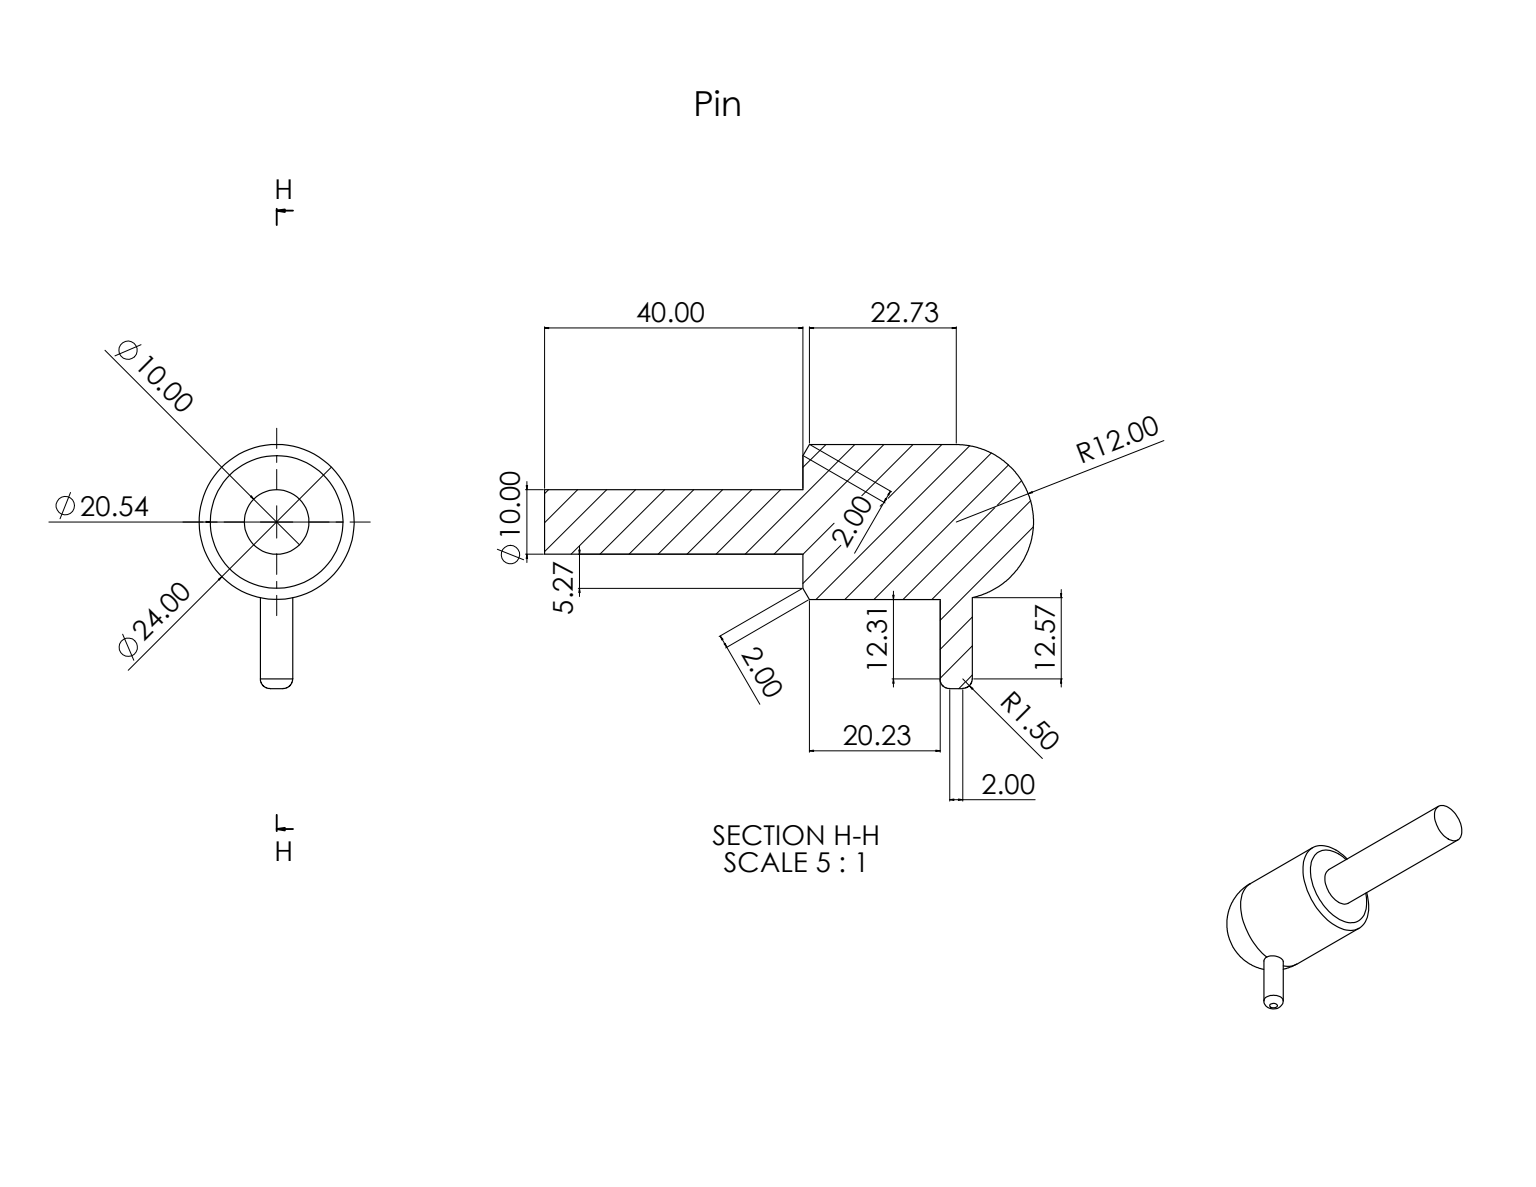
ISO-10303-21;
HEADER;
FILE_DESCRIPTION (('STEP AP214'),
    '1' );
FILE_NAME ('Pin.step',
    '2026-10-26T22:46:44',
    ( '' ),
    ( '' ),
    'SwSTEP 2.0',
    'SolidWorks 2025',
    '' );
FILE_SCHEMA (( 'AUTOMOTIVE_DESIGN' ));
ENDSEC;

DATA;
#9=ORIENTED_EDGE ( 'NONE', *, *, #6510, .F. ) ;
#38=VERTEX_POINT ( 'NONE', #5675 ) ;
#116=DIRECTION ( 'NONE',  ( -0.8660254037844363761, -0.5000000000000043299, 6.872020471724002955E-17 ) ) ;
#132=ORIENTED_EDGE ( 'NONE', *, *, #6398, .F. ) ;
#195=EDGE_CURVE ( 'NONE', #20338, #18465, #2729, .T. ) ;
#229=DIRECTION ( 'NONE',  ( -0.5000000000000046629, 0.8660254037844360431, -0.000000000000000000 ) ) ;
#280=EDGE_LOOP ( 'NONE', ( #9635, #17921, #8883, #13281 ) ) ;
#349=AXIS2_PLACEMENT_3D ( 'NONE', #19014, #17316, #10832 ) ;
#381=ORIENTED_EDGE ( 'NONE', *, *, #17715, .T. ) ;
#391=CIRCLE ( 'NONE', #14642, 12.00000000000002665 ) ;
#499=CARTESIAN_POINT ( 'NONE',  ( 105.1989074543211871, 189.2062061502930135, 11.00000000000001066 ) ) ;
#500=CARTESIAN_POINT ( 'NONE',  ( 97.86136863954072851, 199.4073499008320027, 8.831051211850477145 ) ) ;
#557=ADVANCED_FACE ( 'NONE', ( #8943 ), #5256, .T. ) ;
#571=( NAMED_UNIT ( * ) PLANE_ANGLE_UNIT ( ) SI_UNIT ( $, .RADIAN. ) );
#573=VECTOR ( 'NONE', #13152, 1000.000000000000000 ) ;
#597=DIRECTION ( 'NONE',  ( 0.5000000000000046629, -0.8660254037844360431, 0.000000000000000000 ) ) ;
#619=VECTOR ( 'NONE', #4263, 1000.000000000000114 ) ;
#670=DIRECTION ( 'NONE',  ( 0.8660254037844362651, 0.5000000000000042188, -6.872020471724000490E-17 ) ) ;
#680=AXIS2_PLACEMENT_3D ( 'NONE', #1042, #9181, #2945 ) ;
#733=ORIENTED_EDGE ( 'NONE', *, *, #2224, .T. ) ;
#738=ORIENTED_EDGE ( 'NONE', *, *, #7937, .F. ) ;
#748=AXIS2_PLACEMENT_3D ( 'NONE', #7309, #8909, #2142 ) ;
#770=VECTOR ( 'NONE', #5873, 1000.000000000000000 ) ;
#808=CARTESIAN_POINT ( 'NONE',  ( 96.97892280296886724, 198.7003685781201057, 10.19262075797938749 ) ) ;
#850=CARTESIAN_POINT ( 'NONE',  ( 93.04593889385130012, 210.2557651598135351, 11.00000000000001066 ) ) ;
#883=FACE_BOUND ( 'NONE', #17859, .T. ) ;
#886=DIRECTION ( 'NONE',  ( 0.5000000000000045519, -0.8660254037844359321, 0.000000000000000000 ) ) ;
#911=CARTESIAN_POINT ( 'NONE',  ( 98.22805148513273821, 199.6643403035069753, 8.628462948306966140 ) ) ;
#938=EDGE_LOOP ( 'NONE', ( #1013, #381, #3588, #9, #15721 ) ) ;
#1013=ORIENTED_EDGE ( 'NONE', *, *, #3059, .T. ) ;
#1042=CARTESIAN_POINT ( 'NONE',  ( 106.0649328581056210, 189.7062061502930135, 11.00000000000001066 ) ) ;
#1091=CARTESIAN_POINT ( 'NONE',  ( 105.9489074543212013, 187.9071680446163555, 11.00000000000001066 ) ) ;
#1274=DIRECTION ( 'NONE',  ( 0.000000000000000000, 0.000000000000000000, 1.000000000000000000 ) ) ;
#1345=VERTEX_POINT ( 'NONE', #2130 ) ;
#1356=CARTESIAN_POINT ( 'NONE',  ( 96.89336873520835525, 198.6246579379146340, 11.32949238779788637 ) ) ;
#1392=ORIENTED_EDGE ( 'NONE', *, *, #8590, .F. ) ;
#1422=ORIENTED_EDGE ( 'NONE', *, *, #8317, .T. ) ;
#1435=ORIENTED_EDGE ( 'NONE', *, *, #6398, .T. ) ;
#1450=ADVANCED_FACE ( 'NONE', ( #16963 ), #5914, .T. ) ;
#1455=VERTEX_POINT ( 'NONE', #2551 ) ;
#1460=CARTESIAN_POINT ( 'NONE',  ( 98.91428619100412334, 200.0914894846854679, 13.49999999999996803 ) ) ;
#1469=DIRECTION ( 'NONE',  ( 0.5000000000000046629, -0.8660254037844360431, 0.000000000000000000 ) ) ;
#1562=CARTESIAN_POINT ( 'NONE',  ( 97.35757311143078141, 199.0198733241707600, 12.65155119472265710 ) ) ;
#1569=ORIENTED_EDGE ( 'NONE', *, *, #8317, .F. ) ;
#1666=CARTESIAN_POINT ( 'NONE',  ( 73.36131599811851345, 198.8908428320658288, 11.00000000000001066 ) ) ;
#1667=CARTESIAN_POINT ( 'NONE',  ( 98.62918417965860840, 199.9227537566937940, 13.48335911653028596 ) ) ;
#1681=ORIENTED_EDGE ( 'NONE', *, *, #3937, .T. ) ;
#1704=MECHANICAL_DESIGN_GEOMETRIC_PRESENTATION_REPRESENTATION('',(#5407),#9480);
#1731=AXIS2_PLACEMENT_3D ( 'NONE', #16410, #12923, #9813 ) ;
#1929=CARTESIAN_POINT ( 'NONE',  ( 67.36131599811849924, 207.2831476774790076, 11.00000000000001066 ) ) ;
#2004=DIRECTION ( 'NONE',  ( -0.8660254037844380415, -0.5000000000000008882, 0.000000000000000000 ) ) ;
#2024=DIRECTION ( 'NONE',  ( 0.5000000000000044409, -0.8660254037844360431, 0.000000000000000000 ) ) ;
#2072=AXIS2_PLACEMENT_3D ( 'NONE', #14737, #11324, #13027 ) ;
#2086=CARTESIAN_POINT ( 'NONE',  ( 98.36082807960120533, 199.7525165975381469, 8.580140356014970493 ) ) ;
#2130=CARTESIAN_POINT ( 'NONE',  ( 74.99529059433412215, 194.0607158131436165, 11.00000000000001066 ) ) ;
#2142=DIRECTION ( 'NONE',  ( 0.5000000000000047740, -0.8660254037844359321, 0.000000000000000000 ) ) ;
#2181=AXIS2_PLACEMENT_3D ( 'NONE', #850, #7300, #2761 ) ;
#2224=EDGE_CURVE ( 'NONE', #13549, #1455, #17632, .T. ) ;
#2258=DIRECTION ( 'NONE',  ( -0.8660254037844363761, -0.5000000000000043299, 6.872020471724002955E-17 ) ) ;
#2370=DIRECTION ( 'NONE',  ( -0.8660254037844363761, -0.5000000000000043299, 6.872020471724002955E-17 ) ) ;
#2531=ADVANCED_FACE ( 'NONE', ( #3362 ), #12924, .T. ) ;
#2551=CARTESIAN_POINT ( 'NONE',  ( 77.62926519054968821, 189.4985379866525648, 11.00000000000001066 ) ) ;
#2596=VERTEX_POINT ( 'NONE', #16411 ) ;
#2718=LINE ( 'NONE', #18403, #770 ) ;
#2729=LINE ( 'NONE', #17243, #19805 ) ;
#2757=TOROIDAL_SURFACE ( 'NONE', #11894, 0.9999999999999974465, 1.500000000000000000 ) ;
#2761=DIRECTION ( 'NONE',  ( 0.5000000000000039968, -0.8660254037844362651, 0.000000000000000000 ) ) ;
#2793=AXIS2_PLACEMENT_3D ( 'NONE', #10566, #15166, #13557 ) ;
#2824=DIRECTION ( 'NONE',  ( -0.8660254037844380415, -0.5000000000000008882, 0.000000000000000000 ) ) ;
#2902=FACE_OUTER_BOUND ( 'NONE', #938, .T. ) ;
#2909=DIRECTION ( 'NONE',  ( 0.5000000000000046629, -0.8660254037844360431, 0.000000000000000000 ) ) ;
#2945=DIRECTION ( 'NONE',  ( -1.000000000000000000, 0.000000000000000000, 0.000000000000000000 ) ) ;
#2954=ORIENTED_EDGE ( 'NONE', *, *, #13976, .T. ) ;
#3029=CARTESIAN_POINT ( 'NONE',  ( 98.91428619100412334, 200.0914894846854679, 8.500000000000049738 ) ) ;
#3038=AXIS2_PLACEMENT_3D ( 'NONE', #9596, #11629, #9905 ) ;
#3059=EDGE_CURVE ( 'NONE', #13220, #13875, #391, .T. ) ;
#3151=CARTESIAN_POINT ( 'NONE',  ( 97.07523654288182513, 198.7838771924956518, 12.10917801131580163 ) ) ;
#3155=CARTESIAN_POINT ( 'NONE',  ( 101.0793497004652863, 201.3414894846855248, 11.00000000000001066 ) ) ;
#3221=FACE_OUTER_BOUND ( 'NONE', #4011, .T. ) ;
#3246=CARTESIAN_POINT ( 'NONE',  ( 97.54126021093399856, 199.1658384139430495, 12.88365451894100389 ) ) ;
#3352=CARTESIAN_POINT ( 'NONE',  ( 96.97854020012087517, 198.7000365498672920, 11.80616005232970345 ) ) ;
#3362=FACE_OUTER_BOUND ( 'NONE', #13334, .T. ) ;
#3376=ORIENTED_EDGE ( 'NONE', *, *, #13981, .T. ) ;
#3399=DIRECTION ( 'NONE',  ( 0.8660254037844380415, 0.5000000000000008882, 0.000000000000000000 ) ) ;
#3422=EDGE_CURVE ( 'NONE', #1455, #2596, #2718, .T. ) ;
#3504=DIRECTION ( 'NONE',  ( 0.8660254037844360431, 0.5000000000000045519, 0.000000000000000000 ) ) ;
#3557=CARTESIAN_POINT ( 'NONE',  ( 72.49529059433406530, 198.3908428320658288, 11.00000000000001066 ) ) ;
#3588=ORIENTED_EDGE ( 'NONE', *, *, #12543, .T. ) ;
#3632=CARTESIAN_POINT ( 'NONE',  ( 69.99529059433403688, 202.7209698509880411, 11.00000000000001066 ) ) ;
#3738=DIRECTION ( 'NONE',  ( 0.5000000000000047740, -0.8660254037844359321, 0.000000000000000000 ) ) ;
#3811=MANIFOLD_SOLID_BREP ( 'Chamfer2', #17459 ) ;
#3819=VERTEX_POINT ( 'NONE', #18382 ) ;
#3860=EDGE_CURVE ( 'NONE', #6967, #13875, #6093, .T. ) ;
#3872=CARTESIAN_POINT ( 'NONE',  ( 98.63149783568741213, 199.9241707403680834, 8.516312532717298822 ) ) ;
#3937=EDGE_CURVE ( 'NONE', #18465, #13223, #17962, .T. ) ;
#3956=DIRECTION ( 'NONE',  ( 0.8660254037844380415, 0.5000000000000008882, 0.000000000000000000 ) ) ;
#3984=DIRECTION ( 'NONE',  ( -0.8660254037844361541, -0.5000000000000042188, 6.872020471724001723E-17 ) ) ;
#4011=EDGE_LOOP ( 'NONE', ( #7091, #9421, #18763, #7287 ) ) ;
#4028=CARTESIAN_POINT ( 'NONE',  ( 73.36131599811851345, 198.8908428320658288, 11.00000000000001066 ) ) ;
#4062=ORIENTED_EDGE ( 'NONE', *, *, #3059, .F. ) ;
#4063=AXIS2_PLACEMENT_3D ( 'NONE', #11056, #9339, #886 ) ;
#4138=CONICAL_SURFACE ( 'NONE', #12604, 10.26794919243114634, 1.047197551196596965 ) ;
#4263=DIRECTION ( 'NONE',  ( -0.8660254037844362651, -0.5000000000000042188, 6.872020471724002955E-17 ) ) ;
#4331=AXIS2_PLACEMENT_3D ( 'NONE', #18797, #670, #19952 ) ;
#4359=VERTEX_POINT ( 'NONE', #3155 ) ;
#4366=LINE ( 'NONE', #18896, #619 ) ;
#4402=CIRCLE ( 'NONE', #6404, 5.000000000000039968 ) ;
#4417=AXIS2_PLACEMENT_3D ( 'NONE', #10195, #16577, #3956 ) ;
#4590=DIRECTION ( 'NONE',  ( -0.8660254037844363761, -0.5000000000000043299, 6.872020471724002955E-17 ) ) ;
#4591=FACE_OUTER_BOUND ( 'NONE', #12229, .T. ) ;
#4660=CARTESIAN_POINT ( 'NONE',  ( 98.91428619100422281, 200.0914894846855248, 11.00000000000001066 ) ) ;
#4681=CARTESIAN_POINT ( 'NONE',  ( 103.4382437392645642, 216.2557651598135919, 11.00000000000001066 ) ) ;
#4910=DIRECTION ( 'NONE',  ( 0.8660254037844360431, 0.5000000000000045519, 0.000000000000000000 ) ) ;
#4997=EDGE_CURVE ( 'NONE', #11555, #17136, #5615, .T. ) ;
#5036=DIRECTION ( 'NONE',  ( -0.8660254037844363761, -0.5000000000000043299, 6.872020471724002955E-17 ) ) ;
#5075=AXIS2_PLACEMENT_3D ( 'NONE', #11592, #2258, #15212 ) ;
#5112=EDGE_CURVE ( 'NONE', #1455, #13549, #11532, .T. ) ;
#5132=ORIENTED_EDGE ( 'NONE', *, *, #5112, .T. ) ;
#5166=CARTESIAN_POINT ( 'NONE',  ( 93.04593889385130012, 210.2557651598135351, 11.00000000000000888 ) ) ;
#5185=FACE_OUTER_BOUND ( 'NONE', #16023, .T. ) ;
#5256=TOROIDAL_SURFACE ( 'NONE', #16125, 0.9999999999999974465, 1.500000000000000000 ) ;
#5277=AXIS2_PLACEMENT_3D ( 'NONE', #5556, #3984, #16817 ) ;
#5343=AXIS2_PLACEMENT_3D ( 'NONE', #19222, #20589, #19320 ) ;
#5404=ORIENTED_EDGE ( 'NONE', *, *, #3422, .F. ) ;
#5407=STYLED_ITEM('',(#20988),#3811);
#5445=CARTESIAN_POINT ( 'NONE',  ( 97.26699134085764342, 198.9478798014807808, 9.463061291710214817 ) ) ;
#5500=DIRECTION ( 'NONE',  ( -0.5000000000000043299, 0.8660254037844360431, 0.000000000000000000 ) ) ;
#5556=CARTESIAN_POINT ( 'NONE',  ( 37.85427444295662269, 178.3908428320656299, 11.00000000000001243 ) ) ;
#5576=FACE_OUTER_BOUND ( 'NONE', #13860, .T. ) ;
#5615=LINE ( 'NONE', #12210, #7450 ) ;
#5639=EDGE_CURVE ( 'NONE', #17136, #3819, #6442, .T. ) ;
#5648=( NAMED_UNIT ( * ) PLANE_ANGLE_UNIT ( ) SI_UNIT ( $, .RADIAN. ) );
#5675=CARTESIAN_POINT ( 'NONE',  ( 67.36131599811847082, 209.2831476774790360, 11.00000000000001066 ) ) ;
#5804=ORIENTED_EDGE ( 'NONE', *, *, #195, .F. ) ;
#5824=DIRECTION ( 'NONE',  ( -0.8660254037844362651, -0.5000000000000042188, 6.872020471724002955E-17 ) ) ;
#5837=ORIENTED_EDGE ( 'NONE', *, *, #16586, .T. ) ;
#5864=ADVANCED_FACE ( 'NONE', ( #3221 ), #4138, .T. ) ;
#5873=DIRECTION ( 'NONE',  ( 0.8660254037844417052, -0.4999999999999947820, 1.060575238724906422E-16 ) ) ;
#5914=SPHERICAL_SURFACE ( 'NONE', #2181, 12.00000000000002665 ) ;
#5939=DIRECTION ( 'NONE',  ( 0.5000000000000046629, -0.8660254037844360431, 0.000000000000000000 ) ) ;
#6062=ORIENTED_EDGE ( 'NONE', *, *, #8091, .T. ) ;
#6093=CIRCLE ( 'NONE', #349, 12.00000000000002487 ) ;
#6207=DIRECTION ( 'NONE',  ( 0.8660254037844380415, 0.5000000000000008882, 0.000000000000000000 ) ) ;
#6292=ORIENTED_EDGE ( 'NONE', *, *, #5639, .T. ) ;
#6337=CARTESIAN_POINT ( 'NONE',  ( 87.04593889385124328, 220.6480700052267707, 11.00000000000001066 ) ) ;
#6398=EDGE_CURVE ( 'NONE', #1345, #20338, #18340, .T. ) ;
#6404=AXIS2_PLACEMENT_3D ( 'NONE', #3557, #5036, #14722 ) ;
#6409=DIRECTION ( 'NONE',  ( -0.5000000000000046629, 0.8660254037844360431, -0.000000000000000000 ) ) ;
#6411=CARTESIAN_POINT ( 'NONE',  ( 96.94231704718730214, 198.6680486871722167, 11.65021776913269314 ) ) ;
#6442=CIRCLE ( 'NONE', #1731, 1.500000000000001332 ) ;
#6466=B_SPLINE_CURVE_WITH_KNOTS ( 'NONE', 3,
 ( #7701, #12805, #1356, #6411, #3352, #3151, #16095, #11311, #1562, #3246, #12702, #14307, #16195, #20741, #19060, #1667, #19161, #1460 ),
 .UNSPECIFIED., .F., .F.,
 ( 4, 2, 2, 2, 2, 2, 2, 2, 4 ),
 ( 0.003919784392900028426, 0.004409243773870153045, 0.004898703154840278531, 0.005388162535810403150, 0.005877621916780527769, 0.006367081297750653256, 0.006856540678720777875, 0.007346000059690903361, 0.007835459440661027980 ),
 .UNSPECIFIED. ) ;
#6510=EDGE_CURVE ( 'NONE', #11555, #2596, #12726, .T. ) ;
#6558=CYLINDRICAL_SURFACE ( 'NONE', #7051, 5.000000000000036415 ) ;
#6588=CIRCLE ( 'NONE', #19472, 0.9999999999999917843 ) ;
#6652=DIRECTION ( 'NONE',  ( -0.5000000000000045519, 0.8660254037844359321, 0.000000000000000000 ) ) ;
#6688=ADVANCED_FACE ( 'NONE', ( #13531 ), #2757, .T. ) ;
#6715=VECTOR ( 'NONE', #16730, 1000.000000000000114 ) ;
#6805=EDGE_LOOP ( 'NONE', ( #16956, #13022, #20421, #17398, #20769 ) ) ;
#6825=VECTOR ( 'NONE', #5824, 1000.000000000000114 ) ;
#6967=VERTEX_POINT ( 'NONE', #4681 ) ;
#7051=AXIS2_PLACEMENT_3D ( 'NONE', #8259, #7854, #19304 ) ;
#7091=ORIENTED_EDGE ( 'NONE', *, *, #5112, .F. ) ;
#7098=LINE ( 'NONE', #19815, #10331 ) ;
#7148=EDGE_CURVE ( 'NONE', #17136, #10069, #20322, .T. ) ;
#7154=CARTESIAN_POINT ( 'NONE',  ( 97.97831163141611910, 199.4916918115227702, 8.754184836083465981 ) ) ;
#7258=CARTESIAN_POINT ( 'NONE',  ( 96.89297785063146762, 198.6243099879737599, 10.67381219715677609 ) ) ;
#7270=CARTESIAN_POINT ( 'NONE',  ( 103.0338439448600951, 187.9562061502930135, 11.00000000000001066 ) ) ;
#7287=ORIENTED_EDGE ( 'NONE', *, *, #16586, .F. ) ;
#7300=DIRECTION ( 'NONE',  ( 5.951344303839691563E-17, 3.436010235862028595E-17, 1.000000000000000000 ) ) ;
#7309=CARTESIAN_POINT ( 'NONE',  ( 72.49529059433406530, 198.3908428320658288, 11.00000000000001066 ) ) ;
#7378=( GEOMETRIC_REPRESENTATION_CONTEXT ( 3 ) GLOBAL_UNCERTAINTY_ASSIGNED_CONTEXT ( ( #20801 ) ) GLOBAL_UNIT_ASSIGNED_CONTEXT ( ( #20084, #5648, #15029 ) ) REPRESENTATION_CONTEXT ( 'NONE', 'WORKASPACE' ) );
#7429=AXIS2_PLACEMENT_3D ( 'NONE', #1666, #8005, #12910 ) ;
#7450=VECTOR ( 'NONE', #20360, 1000.000000000000227 ) ;
#7624=CARTESIAN_POINT ( 'NONE',  ( 107.3639709637822648, 190.4562061502930135, 11.00000000000001066 ) ) ;
#7645=DIRECTION ( 'NONE',  ( 0.8660254037844360431, 0.5000000000000045519, 0.000000000000000000 ) ) ;
#7661=ORIENTED_EDGE ( 'NONE', *, *, #7148, .T. ) ;
#7698=DIRECTION ( 'NONE',  ( 0.8660254037844380415, 0.5000000000000008882, 0.000000000000000000 ) ) ;
#7701=CARTESIAN_POINT ( 'NONE',  ( 96.88087538439037871, 198.6134603144003563, 11.00000000000000888 ) ) ;
#7741=EDGE_CURVE ( 'NONE', #10069, #7744, #13554, .T. ) ;
#7744=VERTEX_POINT ( 'NONE', #20740 ) ;
#7802=FACE_OUTER_BOUND ( 'NONE', #6805, .T. ) ;
#7854=DIRECTION ( 'NONE',  ( -0.8660254037844361541, -0.5000000000000042188, 6.872020471724001723E-17 ) ) ;
#7902=EDGE_CURVE ( 'NONE', #20338, #1345, #4402, .T. ) ;
#7937=EDGE_CURVE ( 'NONE', #2596, #38, #20300, .T. ) ;
#7976=EDGE_CURVE ( 'NONE', #6967, #4359, #9123, .T. ) ;
#8005=DIRECTION ( 'NONE',  ( 0.8660254037844360431, 0.5000000000000045519, 0.000000000000000000 ) ) ;
#8091=EDGE_CURVE ( 'NONE', #10891, #11555, #13948, .T. ) ;
#8131=AXIS2_PLACEMENT_3D ( 'NONE', #8265, #229, #3399 ) ;
#8259=CARTESIAN_POINT ( 'NONE',  ( 37.85427444295662269, 178.3908428320656299, 11.00000000000001243 ) ) ;
#8265=CARTESIAN_POINT ( 'NONE',  ( 105.1989074543211728, 189.2062061502930135, 11.00000000000001066 ) ) ;
#8271=ORIENTED_EDGE ( 'NONE', *, *, #13981, .F. ) ;
#8285=EDGE_LOOP ( 'NONE', ( #20903, #12020, #4062, #1422 ) ) ;
#8289=CARTESIAN_POINT ( 'NONE',  ( 72.49529059433407951, 198.3908428320658288, 11.00000000000001066 ) ) ;
#8317=EDGE_CURVE ( 'NONE', #13220, #4359, #9469, .T. ) ;
#8507=ADVANCED_FACE ( 'NONE', ( #10087 ), #19750, .T. ) ;
#8590=EDGE_CURVE ( 'NONE', #13223, #18465, #18287, .T. ) ;
#8644=CARTESIAN_POINT ( 'NONE',  ( 98.77077497239712045, 200.0086332439910279, 8.500000000000021316 ) ) ;
#8650=AXIS2_PLACEMENT_3D ( 'NONE', #12090, #3504, #5500 ) ;
#8687=ADVANCED_FACE ( 'NONE', ( #4591 ), #19016, .T. ) ;
#8732=DIRECTION ( 'NONE',  ( 0.5000000000000038858, -0.8660254037844362651, 0.000000000000000000 ) ) ;
#8746=CARTESIAN_POINT ( 'NONE',  ( 98.91428619100412334, 200.0914894846854679, 13.49999999999996803 ) ) ;
#8883=ORIENTED_EDGE ( 'NONE', *, *, #7741, .T. ) ;
#8899=PRODUCT_DEFINITION_SHAPE ( 'NONE', 'NONE',  #10936 ) ;
#8909=DIRECTION ( 'NONE',  ( -0.8660254037844363761, -0.5000000000000043299, 6.872020471724002955E-17 ) ) ;
#8932=( LENGTH_UNIT ( ) NAMED_UNIT ( * ) SI_UNIT ( .MILLI., .METRE. ) );
#8943=FACE_OUTER_BOUND ( 'NONE', #280, .T. ) ;
#9095=PLANE ( 'NONE',  #17863 ) ;
#9123=CIRCLE ( 'NONE', #3038, 12.00000000000002487 ) ;
#9127=CARTESIAN_POINT ( 'NONE',  ( 40.35427444295665822, 174.0607158131434176, 11.00000000000001243 ) ) ;
#9139=AXIS2_PLACEMENT_3D ( 'NONE', #13619, #2370, #3738 ) ;
#9181=DIRECTION ( 'NONE',  ( 0.000000000000000000, 0.000000000000000000, -1.000000000000000000 ) ) ;
#9236=CARTESIAN_POINT ( 'NONE',  ( 37.85427444295662269, 178.3908428320656299, 11.00000000000001243 ) ) ;
#9280=CARTESIAN_POINT ( 'NONE',  ( 105.1989074543211728, 189.2062061502930135, 11.00000000000001066 ) ) ;
#9339=DIRECTION ( 'NONE',  ( -0.8660254037844361541, -0.5000000000000042188, 6.872020471724001723E-17 ) ) ;
#9351=UNCERTAINTY_MEASURE_WITH_UNIT (LENGTH_MEASURE( 1.000000000000000082E-05 ), #8932, 'distance_accuracy_value', 'NONE');
#9421=ORIENTED_EDGE ( 'NONE', *, *, #3422, .T. ) ;
#9469=CIRCLE ( 'NONE', #19640, 2.499999999999997780 ) ;
#9480=( GEOMETRIC_REPRESENTATION_CONTEXT ( 3 ) GLOBAL_UNCERTAINTY_ASSIGNED_CONTEXT ( ( #9351 ) ) GLOBAL_UNIT_ASSIGNED_CONTEXT ( ( #8932, #571, #12122 ) ) REPRESENTATION_CONTEXT ( 'NONE', 'WORKASPACE' ) );
#9596=CARTESIAN_POINT ( 'NONE',  ( 93.04593889385130012, 210.2557651598135351, 11.00000000000001066 ) ) ;
#9635=ORIENTED_EDGE ( 'NONE', *, *, #5639, .F. ) ;
#9672=AXIS2_PLACEMENT_3D ( 'NONE', #4660, #14541, #2004 ) ;
#9676=DIRECTION ( 'NONE',  ( -0.5000000000000043299, 0.8660254037844360431, 0.000000000000000000 ) ) ;
#9782=ORIENTED_EDGE ( 'NONE', *, *, #7741, .F. ) ;
#9795=ORIENTED_EDGE ( 'NONE', *, *, #3860, .F. ) ;
#9806=CYLINDRICAL_SURFACE ( 'NONE', #5277, 5.000000000000036415 ) ;
#9813=DIRECTION ( 'NONE',  ( 1.000000000000000000, 0.000000000000000000, 0.000000000000000000 ) ) ;
#9855=CIRCLE ( 'NONE', #14973, 0.9999999999999917843 ) ;
#9905=DIRECTION ( 'NONE',  ( -1.000000000000000000, 0.000000000000000000, 0.000000000000000000 ) ) ;
#9948=EDGE_LOOP ( 'NONE', ( #19226, #6292, #11319, #9782 ) ) ;
#10069=VERTEX_POINT ( 'NONE', #7624 ) ;
#10087=FACE_OUTER_BOUND ( 'NONE', #12180, .T. ) ;
#10109=DIRECTION ( 'NONE',  ( 0.8660254037844359321, 0.5000000000000046629, 0.000000000000000000 ) ) ;
#10195=CARTESIAN_POINT ( 'NONE',  ( 94.31531706421118599, 208.0571376747316492, 11.00000000000001066 ) ) ;
#10331=VECTOR ( 'NONE', #2024, 1000.000000000000227 ) ;
#10344=CIRCLE ( 'NONE', #9672, 2.499999999999997780 ) ;
#10370=ADVANCED_FACE ( 'NONE', ( #5576 ), #15061, .T. ) ;
#10420=SHAPE_REPRESENTATION_RELATIONSHIP ( 'NONE' , 'NONE' ,  #14136, #12645 ) ;
#10456=EDGE_LOOP ( 'NONE', ( #733, #5132 ) ) ;
#10566=CARTESIAN_POINT ( 'NONE',  ( 105.9489074543212013, 187.9071680446163555, 11.00000000000001066 ) ) ;
#10643=DIRECTION ( 'NONE',  ( -0.5000000000000037748, 0.8660254037844364872, 0.000000000000000000 ) ) ;
#10653=DIRECTION ( 'NONE',  ( -0.8660254037844362651, -0.5000000000000042188, 6.872020471724002955E-17 ) ) ;
#10832=DIRECTION ( 'NONE',  ( 1.000000000000000000, 0.000000000000000000, -1.445602896647336205E-16 ) ) ;
#10891=VERTEX_POINT ( 'NONE', #3029 ) ;
#10936=PRODUCT_DEFINITION ( 'UNKNOWN', '', #18249, #14271 ) ;
#11028=CARTESIAN_POINT ( 'NONE',  ( 43.85427444295667954, 167.9985379866523942, 11.00000000000001243 ) ) ;
#11051=AXIS2_PLACEMENT_3D ( 'NONE', #5166, #18219, #18017 ) ;
#11056=CARTESIAN_POINT ( 'NONE',  ( 37.85427444295662269, 178.3908428320656299, 11.00000000000001243 ) ) ;
#11264=CIRCLE ( 'NONE', #17700, 12.00000000000000178 ) ;
#11270=DIRECTION ( 'NONE',  ( 0.5000000000000047740, -0.8660254037844359321, 0.000000000000000000 ) ) ;
#11311=CARTESIAN_POINT ( 'NONE',  ( 97.27623782526788432, 198.9531532459614880, 12.52486517255494824 ) ) ;
#11319=ORIENTED_EDGE ( 'NONE', *, *, #14796, .F. ) ;
#11324=DIRECTION ( 'NONE',  ( 5.951344303839691563E-17, 3.436010235862028595E-17, 1.000000000000000000 ) ) ;
#11352=FACE_OUTER_BOUND ( 'NONE', #15794, .T. ) ;
#11445=EDGE_CURVE ( 'NONE', #3819, #7744, #9855, .T. ) ;
#11532=CIRCLE ( 'NONE', #16270, 10.26794919243111437 ) ;
#11555=VERTEX_POINT ( 'NONE', #16409 ) ;
#11592=CARTESIAN_POINT ( 'NONE',  ( 72.49529059433409373, 198.3908428320658004, 11.00000000000001066 ) ) ;
#11629=DIRECTION ( 'NONE',  ( -5.951344303839690331E-17, -3.436010235862032909E-17, -1.000000000000000000 ) ) ;
#11690=ORIENTED_EDGE ( 'NONE', *, *, #4997, .T. ) ;
#11791=ORIENTED_EDGE ( 'NONE', *, *, #7937, .T. ) ;
#11894=AXIS2_PLACEMENT_3D ( 'NONE', #499, #597, #10109 ) ;
#11927=CARTESIAN_POINT ( 'NONE',  ( 93.04593889385130012, 210.2557651598135351, 11.00000000000000888 ) ) ;
#11945=CARTESIAN_POINT ( 'NONE',  ( 96.88087538439039292, 198.6134603144004132, 10.83638872456144675 ) ) ;
#11963=CIRCLE ( 'NONE', #14686, 2.499999999999997780 ) ;
#11975=AXIS2_PLACEMENT_3D ( 'NONE', #14304, #20739, #6207 ) ;
#12020=ORIENTED_EDGE ( 'NONE', *, *, #3860, .T. ) ;
#12031=DIRECTION ( 'NONE',  ( -0.8660254037844363761, -0.5000000000000043299, 6.872020471724002955E-17 ) ) ;
#12090=CARTESIAN_POINT ( 'NONE',  ( 72.49529059433407951, 198.3908428320658288, 11.00000000000001066 ) ) ;
#12120=FACE_OUTER_BOUND ( 'NONE', #10456, .T. ) ;
#12122=( NAMED_UNIT ( * ) SI_UNIT ( $, .STERADIAN. ) SOLID_ANGLE_UNIT ( ) );
#12180=EDGE_LOOP ( 'NONE', ( #18941, #11690, #7661, #19069, #1569 ) ) ;
#12188=DIRECTION ( 'NONE',  ( -0.5000000000000042188, 0.8660254037844362651, 0.000000000000000000 ) ) ;
#12210=CARTESIAN_POINT ( 'NONE',  ( 92.15025355475009405, 206.8071376747316492, 11.00000000000001066 ) ) ;
#12229=EDGE_LOOP ( 'NONE', ( #17533, #3376, #6062, #13729, #11791 ) ) ;
#12248=DIRECTION ( 'NONE',  ( 0.8660254037844359321, 0.5000000000000046629, 0.000000000000000000 ) ) ;
#12308=FACE_OUTER_BOUND ( 'NONE', #15169, .T. ) ;
#12543=EDGE_CURVE ( 'NONE', #38, #2596, #11264, .T. ) ;
#12604=AXIS2_PLACEMENT_3D ( 'NONE', #8289, #4910, #9676 ) ;
#12645=ADVANCED_BREP_SHAPE_REPRESENTATION ( '', ( #3811, #18233 ), #7378 ) ;
#12702=CARTESIAN_POINT ( 'NONE',  ( 97.64153595007269359, 199.2434332111931212, 12.98669150848017573 ) ) ;
#12726=LINE ( 'NONE', #11028, #6825 ) ;
#12736=SHAPE_DEFINITION_REPRESENTATION ( #8899, #14136 ) ;
#12805=CARTESIAN_POINT ( 'NONE',  ( 96.88087538439037871, 198.6134603144003847, 11.16343975192298466 ) ) ;
#12864=CYLINDRICAL_SURFACE ( 'NONE', #5343, 11.99999999999999822 ) ;
#12910=DIRECTION ( 'NONE',  ( -0.5000000000000049960, 0.8660254037844357100, 0.000000000000000000 ) ) ;
#12923=DIRECTION ( 'NONE',  ( 1.060575238724903710E-16, 6.123233995736822735E-17, 1.000000000000000000 ) ) ;
#12924=SPHERICAL_SURFACE ( 'NONE', #2072, 12.00000000000002665 ) ;
#12981=ORIENTED_EDGE ( 'NONE', *, *, #18965, .F. ) ;
#13022=ORIENTED_EDGE ( 'NONE', *, *, #8091, .F. ) ;
#13027=DIRECTION ( 'NONE',  ( 0.5000000000000039968, -0.8660254037844362651, 0.000000000000000000 ) ) ;
#13036=EDGE_CURVE ( 'NONE', #10069, #17136, #11963, .T. ) ;
#13131=ADVANCED_FACE ( 'NONE', ( #7802 ), #14403, .T. ) ;
#13152=DIRECTION ( 'NONE',  ( -4.385380947269368335E-15, 1.000000000000000000, 0.000000000000000000 ) ) ;
#13220=VERTEX_POINT ( 'NONE', #8746 ) ;
#13223=VERTEX_POINT ( 'NONE', #9127 ) ;
#13281=ORIENTED_EDGE ( 'NONE', *, *, #11445, .F. ) ;
#13334=EDGE_LOOP ( 'NONE', ( #9795, #19554, #2954, #8271 ) ) ;
#13357=ORIENTED_EDGE ( 'NONE', *, *, #195, .T. ) ;
#13410=CIRCLE ( 'NONE', #11051, 12.00000000000002665 ) ;
#13430=CARTESIAN_POINT ( 'NONE',  ( 97.12292291349348261, 198.8252231143156621, 9.741427369672765124 ) ) ;
#13531=FACE_OUTER_BOUND ( 'NONE', #9948, .T. ) ;
#13549=VERTEX_POINT ( 'NONE', #1929 ) ;
#13554=CIRCLE ( 'NONE', #680, 1.500000000000001332 ) ;
#13557=DIRECTION ( 'NONE',  ( 0.8660254037844360431, 0.5000000000000045519, 0.000000000000000000 ) ) ;
#13617=ORIENTED_EDGE ( 'NONE', *, *, #3937, .F. ) ;
#13619=CARTESIAN_POINT ( 'NONE',  ( 37.85427444295662269, 178.3908428320656299, 11.00000000000001243 ) ) ;
#13729=ORIENTED_EDGE ( 'NONE', *, *, #6510, .T. ) ;
#13777=ORIENTED_EDGE ( 'NONE', *, *, #7902, .T. ) ;
#13838=CARTESIAN_POINT ( 'NONE',  ( 105.1989074543211871, 189.2062061502930135, 11.00000000000001066 ) ) ;
#13860=EDGE_LOOP ( 'NONE', ( #19427, #19139 ) ) ;
#13875=VERTEX_POINT ( 'NONE', #6337 ) ;
#13948=B_SPLINE_CURVE_WITH_KNOTS ( 'NONE', 3,
 ( #16599, #8644, #3872, #2086, #911, #7154, #500, #19984, #15041, #5445, #13430, #808, #15247, #7258, #11945, #18404 ),
 .UNSPECIFIED., .F., .F.,
 ( 4, 2, 2, 2, 2, 2, 2, 4 ),
 ( 1.398578778534940505E-17, 0.0004899730491125216594, 0.0009799460982250292242, 0.001469919147337537006, 0.001959892196450044571, 0.002939838294675023271, 0.003429811343787525849, 0.003919784392900028426 ),
 .UNSPECIFIED. ) ;
#13976=EDGE_CURVE ( 'NONE', #4359, #10891, #10344, .T. ) ;
#13981=EDGE_CURVE ( 'NONE', #13875, #10891, #13410, .T. ) ;
#14096=APPLICATION_CONTEXT ( 'automotive_design' ) ;
#14136=SHAPE_REPRESENTATION ( 'Pin', ( #18233 ), #7378 ) ;
#14271=PRODUCT_DEFINITION_CONTEXT ( 'detailed design', #14096, 'design' ) ;
#14304=CARTESIAN_POINT ( 'NONE',  ( 94.31531706421118599, 208.0571376747316492, 11.00000000000001066 ) ) ;
#14306=EDGE_CURVE ( 'NONE', #11555, #13220, #6466, .T. ) ;
#14307=CARTESIAN_POINT ( 'NONE',  ( 97.85954905003006843, 199.4060149184856243, 13.16759434796133554 ) ) ;
#14403=CYLINDRICAL_SURFACE ( 'NONE', #11975, 2.499999999999997780 ) ;
#14415=ORIENTED_EDGE ( 'NONE', *, *, #2224, .F. ) ;
#14416=CARTESIAN_POINT ( 'NONE',  ( 105.9489074543212013, 187.9071680446163555, 11.00000000000001066 ) ) ;
#14484=ADVANCED_FACE ( 'NONE', ( #18405 ), #9806, .T. ) ;
#14541=DIRECTION ( 'NONE',  ( -0.5000000000000037748, 0.8660254037844364872, 0.000000000000000000 ) ) ;
#14548=CARTESIAN_POINT ( 'NONE',  ( 72.49529059433409373, 198.3908428320658004, 11.00000000000001066 ) ) ;
#14642=AXIS2_PLACEMENT_3D ( 'NONE', #11927, #12031, #8732 ) ;
#14686=AXIS2_PLACEMENT_3D ( 'NONE', #9280, #6409, #7698 ) ;
#14722=DIRECTION ( 'NONE',  ( 0.5000000000000047740, -0.8660254037844359321, 0.000000000000000000 ) ) ;
#14737=CARTESIAN_POINT ( 'NONE',  ( 93.04593889385130012, 210.2557651598135351, 11.00000000000001066 ) ) ;
#14796=EDGE_CURVE ( 'NONE', #7744, #3819, #6588, .T. ) ;
#14902=ORIENTED_EDGE ( 'NONE', *, *, #8590, .T. ) ;
#14973=AXIS2_PLACEMENT_3D ( 'NONE', #14416, #1469, #20845 ) ;
#15029=( NAMED_UNIT ( * ) SI_UNIT ( $, .STERADIAN. ) SOLID_ANGLE_UNIT ( ) );
#15041=CARTESIAN_POINT ( 'NONE',  ( 97.53995344223362451, 199.1648067970725720, 9.117919383928111188 ) ) ;
#15061=PLANE ( 'NONE',  #2793 ) ;
#15078=LINE ( 'NONE', #16642, #573 ) ;
#15164=LINE ( 'NONE', #19791, #6715 ) ;
#15166=DIRECTION ( 'NONE',  ( 0.5000000000000045519, -0.8660254037844360431, 0.000000000000000000 ) ) ;
#15169=EDGE_LOOP ( 'NONE', ( #14902, #1681 ) ) ;
#15212=DIRECTION ( 'NONE',  ( -0.5000000000000045519, 0.8660254037844359321, 0.000000000000000000 ) ) ;
#15247=CARTESIAN_POINT ( 'NONE',  ( 96.94205509780233854, 198.6678179064276435, 10.35076502982056113 ) ) ;
#15721=ORIENTED_EDGE ( 'NONE', *, *, #14306, .T. ) ;
#15763=CARTESIAN_POINT ( 'NONE',  ( 98.91428619100422281, 200.0914894846855248, 11.00000000000001066 ) ) ;
#15794=EDGE_LOOP ( 'NONE', ( #1435, #13357, #1392, #12981 ) ) ;
#15903=CARTESIAN_POINT ( 'NONE',  ( 0.000000000000000000, 0.000000000000000000, 0.000000000000000000 ) ) ;
#16023=EDGE_LOOP ( 'NONE', ( #5404, #14415, #5837, #738 ) ) ;
#16095=CARTESIAN_POINT ( 'NONE',  ( 97.13553065963888855, 198.8355456815907303, 12.25473482689746696 ) ) ;
#16125=AXIS2_PLACEMENT_3D ( 'NONE', #13838, #2909, #12248 ) ;
#16195=CARTESIAN_POINT ( 'NONE',  ( 97.97877128586738138, 199.4920122637983297, 13.24606046902644074 ) ) ;
#16270=AXIS2_PLACEMENT_3D ( 'NONE', #14548, #116, #6652 ) ;
#16409=CARTESIAN_POINT ( 'NONE',  ( 96.88087538439037871, 198.6134603144003563, 11.00000000000000888 ) ) ;
#16410=CARTESIAN_POINT ( 'NONE',  ( 104.3328820505367531, 188.7062061502930135, 11.00000000000001066 ) ) ;
#16411=CARTESIAN_POINT ( 'NONE',  ( 79.36131599811857029, 188.4985379866525932, 11.00000000000001066 ) ) ;
#16577=DIRECTION ( 'NONE',  ( 0.5000000000000045519, -0.8660254037844361541, 0.000000000000000000 ) ) ;
#16586=EDGE_CURVE ( 'NONE', #13549, #38, #15078, .T. ) ;
#16599=CARTESIAN_POINT ( 'NONE',  ( 98.91428619100412334, 200.0914894846854679, 8.500000000000049738 ) ) ;
#16642=CARTESIAN_POINT ( 'NONE',  ( 67.36131599811847082, 207.2831476774790644, 11.00000000000001066 ) ) ;
#16649=CARTESIAN_POINT ( 'NONE',  ( 35.35427444295658717, 182.7209698509878422, 11.00000000000001243 ) ) ;
#16681=ADVANCED_FACE ( 'NONE', ( #12308 ), #9095, .F. ) ;
#16730=DIRECTION ( 'NONE',  ( -0.8660254037844362651, -0.5000000000000042188, 6.872020471724002955E-17 ) ) ;
#16817=DIRECTION ( 'NONE',  ( 0.5000000000000037748, -0.8660254037844364872, 0.000000000000000000 ) ) ;
#16956=ORIENTED_EDGE ( 'NONE', *, *, #4997, .F. ) ;
#16963=FACE_OUTER_BOUND ( 'NONE', #8285, .T. ) ;
#17072=DIRECTION ( 'NONE',  ( 0.8660254037844362651, 0.5000000000000042188, -6.872020471724000490E-17 ) ) ;
#17136=VERTEX_POINT ( 'NONE', #7270 ) ;
#17243=CARTESIAN_POINT ( 'NONE',  ( 35.35427444295658717, 182.7209698509878422, 11.00000000000001243 ) ) ;
#17282=AXIS2_PLACEMENT_3D ( 'NONE', #9236, #4590, #11270 ) ;
#17316=DIRECTION ( 'NONE',  ( 1.207457829957650937E-16, -7.169742151387006041E-17, 1.000000000000000000 ) ) ;
#17398=ORIENTED_EDGE ( 'NONE', *, *, #19748, .T. ) ;
#17459=CLOSED_SHELL ( 'NONE', ( #5864, #6688, #8507, #1450, #18083, #18342, #14484, #20544, #8687, #2531, #16681, #13131, #10370, #557, #19732 ) ) ;
#17533=ORIENTED_EDGE ( 'NONE', *, *, #17715, .F. ) ;
#17632=CIRCLE ( 'NONE', #5075, 10.26794919243111437 ) ;
#17700=AXIS2_PLACEMENT_3D ( 'NONE', #4028, #20242, #18664 ) ;
#17715=EDGE_CURVE ( 'NONE', #13875, #38, #4366, .T. ) ;
#17859=EDGE_LOOP ( 'NONE', ( #132, #20252 ) ) ;
#17863=AXIS2_PLACEMENT_3D ( 'NONE', #20231, #17072, #12188 ) ;
#17895=EDGE_LOOP ( 'NONE', ( #5804, #13777, #18922, #13617 ) ) ;
#17921=ORIENTED_EDGE ( 'NONE', *, *, #13036, .F. ) ;
#17962=CIRCLE ( 'NONE', #17282, 5.000000000000039968 ) ;
#18017=DIRECTION ( 'NONE',  ( 0.5000000000000038858, -0.8660254037844362651, 0.000000000000000000 ) ) ;
#18083=ADVANCED_FACE ( 'NONE', ( #2902 ), #12864, .T. ) ;
#18202=PRODUCT ( 'Pin', 'Pin', '', ( #18891 ) ) ;
#18219=DIRECTION ( 'NONE',  ( -0.8660254037844363761, -0.5000000000000043299, 6.872020471724002955E-17 ) ) ;
#18233=AXIS2_PLACEMENT_3D ( 'NONE', #15903, #1274, #19656 ) ;
#18249=PRODUCT_DEFINITION_FORMATION_WITH_SPECIFIED_SOURCE ( 'ANY', '', #18202, .NOT_KNOWN. ) ;
#18287=CIRCLE ( 'NONE', #9139, 5.000000000000039968 ) ;
#18340=CIRCLE ( 'NONE', #748, 5.000000000000039968 ) ;
#18342=ADVANCED_FACE ( 'NONE', ( #11352 ), #6558, .T. ) ;
#18382=CARTESIAN_POINT ( 'NONE',  ( 105.0828820505367531, 187.4071680446163555, 11.00000000000001066 ) ) ;
#18403=CARTESIAN_POINT ( 'NONE',  ( 77.62926519054970242, 189.4985379866525648, 11.00000000000001066 ) ) ;
#18404=CARTESIAN_POINT ( 'NONE',  ( 96.88087538439037871, 198.6134603144003563, 11.00000000000000888 ) ) ;
#18405=FACE_OUTER_BOUND ( 'NONE', #17895, .T. ) ;
#18465=VERTEX_POINT ( 'NONE', #16649 ) ;
#18478=CONICAL_SURFACE ( 'NONE', #8650, 10.26794919243114634, 1.047197551196596965 ) ;
#18664=DIRECTION ( 'NONE',  ( -0.5000000000000049960, 0.8660254037844357100, 0.000000000000000000 ) ) ;
#18695=PLANE ( 'NONE',  #4331 ) ;
#18763=ORIENTED_EDGE ( 'NONE', *, *, #12543, .F. ) ;
#18797=CARTESIAN_POINT ( 'NONE',  ( 69.99529059433403688, 202.7209698509880411, 11.00000000000001066 ) ) ;
#18891=PRODUCT_CONTEXT ( 'NONE', #19729, 'mechanical' ) ;
#18896=CARTESIAN_POINT ( 'NONE',  ( 31.85427444295656940, 188.7831476774788655, 11.00000000000001421 ) ) ;
#18922=ORIENTED_EDGE ( 'NONE', *, *, #18965, .T. ) ;
#18941=ORIENTED_EDGE ( 'NONE', *, *, #14306, .F. ) ;
#18965=EDGE_CURVE ( 'NONE', #1345, #13223, #15164, .T. ) ;
#19014=CARTESIAN_POINT ( 'NONE',  ( 93.04593889385130012, 210.2557651598135351, 11.00000000000001066 ) ) ;
#19016=CYLINDRICAL_SURFACE ( 'NONE', #4063, 11.99999999999999822 ) ;
#19060=CARTESIAN_POINT ( 'NONE',  ( 98.35782272495457335, 199.7505593597859956, 13.41892939600676016 ) ) ;
#19069=ORIENTED_EDGE ( 'NONE', *, *, #19748, .F. ) ;
#19139=ORIENTED_EDGE ( 'NONE', *, *, #11445, .T. ) ;
#19161=CARTESIAN_POINT ( 'NONE',  ( 98.77092417049759376, 200.0087193835544497, 13.49999999999999822 ) ) ;
#19222=CARTESIAN_POINT ( 'NONE',  ( 37.85427444295662269, 178.3908428320656299, 11.00000000000001243 ) ) ;
#19226=ORIENTED_EDGE ( 'NONE', *, *, #7148, .F. ) ;
#19304=DIRECTION ( 'NONE',  ( 0.5000000000000037748, -0.8660254037844364872, 0.000000000000000000 ) ) ;
#19320=DIRECTION ( 'NONE',  ( 0.5000000000000045519, -0.8660254037844359321, 0.000000000000000000 ) ) ;
#19427=ORIENTED_EDGE ( 'NONE', *, *, #14796, .T. ) ;
#19472=AXIS2_PLACEMENT_3D ( 'NONE', #1091, #5939, #7645 ) ;
#19554=ORIENTED_EDGE ( 'NONE', *, *, #7976, .T. ) ;
#19640=AXIS2_PLACEMENT_3D ( 'NONE', #15763, #10643, #2824 ) ;
#19656=DIRECTION ( 'NONE',  ( 1.000000000000000000, 0.000000000000000000, 0.000000000000000000 ) ) ;
#19729=APPLICATION_CONTEXT ( 'automotive_design' ) ;
#19732=ADVANCED_FACE ( 'NONE', ( #5185 ), #18478, .T. ) ;
#19748=EDGE_CURVE ( 'NONE', #4359, #10069, #7098, .T. ) ;
#19750=CYLINDRICAL_SURFACE ( 'NONE', #4417, 2.499999999999997780 ) ;
#19791=CARTESIAN_POINT ( 'NONE',  ( 40.35427444295665822, 174.0607158131434176, 11.00000000000001243 ) ) ;
#19805=VECTOR ( 'NONE', #10653, 1000.000000000000114 ) ;
#19815=CARTESIAN_POINT ( 'NONE',  ( 96.48038057367227793, 209.3071376747316776, 11.00000000000001066 ) ) ;
#19952=DIRECTION ( 'NONE',  ( -0.5000000000000042188, 0.8660254037844362651, 0.000000000000000000 ) ) ;
#19984=CARTESIAN_POINT ( 'NONE',  ( 97.64222899835127123, 199.2439717600714744, 9.012579768282821036 ) ) ;
#20084=( LENGTH_UNIT ( ) NAMED_UNIT ( * ) SI_UNIT ( .MILLI., .METRE. ) );
#20231=CARTESIAN_POINT ( 'NONE',  ( 35.35427444295658006, 182.7209698509878422, 11.00000000000001243 ) ) ;
#20242=DIRECTION ( 'NONE',  ( 0.8660254037844360431, 0.5000000000000045519, 0.000000000000000000 ) ) ;
#20252=ORIENTED_EDGE ( 'NONE', *, *, #7902, .F. ) ;
#20300=CIRCLE ( 'NONE', #7429, 12.00000000000000178 ) ;
#20322=CIRCLE ( 'NONE', #8131, 2.499999999999997780 ) ;
#20338=VERTEX_POINT ( 'NONE', #3632 ) ;
#20360=DIRECTION ( 'NONE',  ( 0.5000000000000044409, -0.8660254037844360431, 0.000000000000000000 ) ) ;
#20421=ORIENTED_EDGE ( 'NONE', *, *, #13976, .F. ) ;
#20544=ADVANCED_FACE ( 'NONE', ( #12120, #883 ), #18695, .F. ) ;
#20589=DIRECTION ( 'NONE',  ( -0.8660254037844361541, -0.5000000000000042188, 6.872020471724001723E-17 ) ) ;
#20739=DIRECTION ( 'NONE',  ( 0.5000000000000045519, -0.8660254037844361541, 0.000000000000000000 ) ) ;
#20740=CARTESIAN_POINT ( 'NONE',  ( 106.8149328581056352, 188.4071680446163555, 11.00000000000001066 ) ) ;
#20741=CARTESIAN_POINT ( 'NONE',  ( 98.22787951438910170, 199.6642187277107041, 13.37143655376591767 ) ) ;
#20769=ORIENTED_EDGE ( 'NONE', *, *, #13036, .T. ) ;
#20801=UNCERTAINTY_MEASURE_WITH_UNIT (LENGTH_MEASURE( 1.000000000000000082E-05 ), #20084, 'distance_accuracy_value', 'NONE');
#20845=DIRECTION ( 'NONE',  ( 0.8660254037844360431, 0.5000000000000045519, 0.000000000000000000 ) ) ;
#20903=ORIENTED_EDGE ( 'NONE', *, *, #7976, .F. ) ;
#20982=COLOUR_RGB('Grey',0.48,0.52,0.57);
#20983=FILL_AREA_STYLE_COLOUR('',#20982);
#20984=FILL_AREA_STYLE('',(#20983));
#20985=SURFACE_STYLE_FILL_AREA(#20984);
#20986=SURFACE_SIDE_STYLE('',(#20985));
#20987=SURFACE_STYLE_USAGE(.BOTH.,#20986);
#20988=PRESENTATION_STYLE_ASSIGNMENT((#20987));
ENDSEC;
END-ISO-10303-21;
